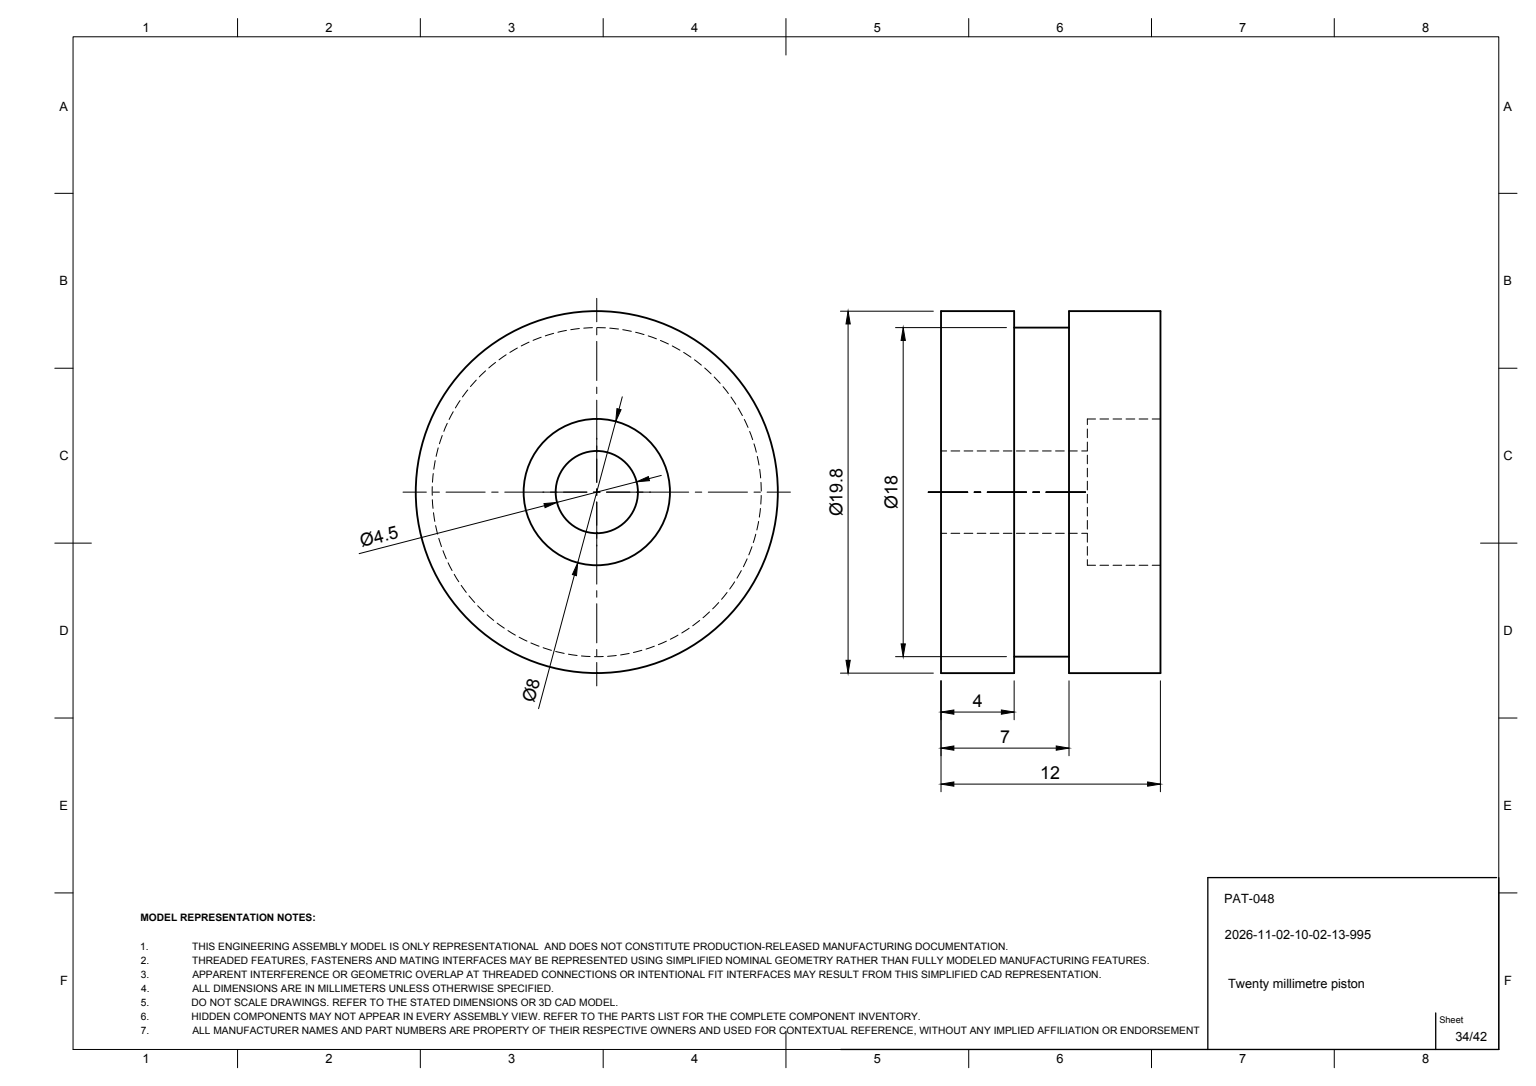
ISO-10303-21;
HEADER;
/* Generated by software containing ST-Developer
 * from STEP Tools, Inc. (www.steptools.com) 
 */

FILE_DESCRIPTION(
/* description */ ('Guided pneumatic stop gate'),
/* implementation_level */ '2;1');

FILE_NAME(
/* name */ 'Twenty millimetre piston.step',
/* time_stamp */ '2026-10-27T21:43:45-07:00',
/* author */ (''),
/* organization */ (''),
/* preprocessor_version */ 'ST-DEVELOPER v20.2',
/* originating_system */ 'Autodesk Translation Framework v15.17.0.0',
/* authorisation */ '');

FILE_SCHEMA (('AUTOMOTIVE_DESIGN { 1 0 10303 214 3 1 1 }'));
ENDSEC;

DATA;
#10=MECHANICAL_DESIGN_GEOMETRIC_PRESENTATION_REPRESENTATION('',(#563),#14392);
#479=SHAPE_REPRESENTATION_RELATIONSHIP('SRR','None',#14616,#521);
#521=ADVANCED_BREP_SHAPE_REPRESENTATION('',(#602),#14378);
#563=STYLED_ITEM('',(#14905),#602);
#602=MANIFOLD_SOLID_BREP('Body1',#7906);
#791=FACE_BOUND('',#2129,.T.);
#792=FACE_BOUND('',#2132,.T.);
#793=FACE_BOUND('',#2134,.T.);
#794=FACE_BOUND('',#2139,.T.);
#795=FACE_BOUND('',#2141,.T.);
#1043=PLANE('',#9159);
#1044=PLANE('',#9164);
#1045=PLANE('',#9166);
#1046=PLANE('',#9174);
#1047=PLANE('',#9175);
#1476=FACE_OUTER_BOUND('',#2127,.T.);
#1477=FACE_OUTER_BOUND('',#2128,.T.);
#1478=FACE_OUTER_BOUND('',#2130,.T.);
#1479=FACE_OUTER_BOUND('',#2131,.T.);
#1480=FACE_OUTER_BOUND('',#2133,.T.);
#1481=FACE_OUTER_BOUND('',#2135,.T.);
#1482=FACE_OUTER_BOUND('',#2136,.T.);
#1483=FACE_OUTER_BOUND('',#2137,.T.);
#1484=FACE_OUTER_BOUND('',#2138,.T.);
#1485=FACE_OUTER_BOUND('',#2140,.T.);
#2127=EDGE_LOOP('',(#6772,#6773,#6774,#6775));
#2128=EDGE_LOOP('',(#6776));
#2129=EDGE_LOOP('',(#6777));
#2130=EDGE_LOOP('',(#6778,#6779,#6780,#6781));
#2131=EDGE_LOOP('',(#6782));
#2132=EDGE_LOOP('',(#6783));
#2133=EDGE_LOOP('',(#6784));
#2134=EDGE_LOOP('',(#6785));
#2135=EDGE_LOOP('',(#6786,#6787,#6788,#6789));
#2136=EDGE_LOOP('',(#6790,#6791,#6792,#6793));
#2137=EDGE_LOOP('',(#6794,#6795,#6796,#6797));
#2138=EDGE_LOOP('',(#6798));
#2139=EDGE_LOOP('',(#6799));
#2140=EDGE_LOOP('',(#6800));
#2141=EDGE_LOOP('',(#6801));
#2686=LINE('',#13608,#3231);
#2687=LINE('',#13617,#3232);
#2688=LINE('',#13627,#3233);
#2689=LINE('',#13631,#3234);
#2690=LINE('',#13636,#3235);
#3231=VECTOR('',#11337,0.4);
#3232=VECTOR('',#11348,0.9);
#3233=VECTOR('',#11361,0.99);
#3234=VECTOR('',#11366,0.225);
#3235=VECTOR('',#11373,0.99);
#3662=CIRCLE('',#9157,0.4);
#3663=CIRCLE('',#9158,0.4);
#3664=CIRCLE('',#9160,0.225);
#3665=CIRCLE('',#9162,0.9);
#3666=CIRCLE('',#9163,0.9);
#3667=CIRCLE('',#9165,0.99);
#3668=CIRCLE('',#9167,0.99);
#3669=CIRCLE('',#9169,0.99);
#3670=CIRCLE('',#9171,0.225);
#3671=CIRCLE('',#9173,0.99);
#4205=VERTEX_POINT('',#13605);
#4206=VERTEX_POINT('',#13607);
#4207=VERTEX_POINT('',#13611);
#4208=VERTEX_POINT('',#13614);
#4209=VERTEX_POINT('',#13616);
#4210=VERTEX_POINT('',#13620);
#4211=VERTEX_POINT('',#13623);
#4212=VERTEX_POINT('',#13626);
#4213=VERTEX_POINT('',#13630);
#4214=VERTEX_POINT('',#13634);
#5084=EDGE_CURVE('',#4205,#4205,#3662,.T.);
#5085=EDGE_CURVE('',#4205,#4206,#2686,.T.);
#5086=EDGE_CURVE('',#4206,#4206,#3663,.T.);
#5087=EDGE_CURVE('',#4207,#4207,#3664,.T.);
#5088=EDGE_CURVE('',#4208,#4208,#3665,.T.);
#5089=EDGE_CURVE('',#4208,#4209,#2687,.T.);
#5090=EDGE_CURVE('',#4209,#4209,#3666,.T.);
#5091=EDGE_CURVE('',#4210,#4210,#3667,.T.);
#5092=EDGE_CURVE('',#4211,#4211,#3668,.T.);
#5093=EDGE_CURVE('',#4211,#4212,#2688,.T.);
#5094=EDGE_CURVE('',#4212,#4212,#3669,.T.);
#5095=EDGE_CURVE('',#4207,#4213,#2689,.T.);
#5096=EDGE_CURVE('',#4213,#4213,#3670,.T.);
#5097=EDGE_CURVE('',#4214,#4214,#3671,.T.);
#5098=EDGE_CURVE('',#4214,#4210,#2690,.T.);
#6772=ORIENTED_EDGE('',*,*,#5084,.F.);
#6773=ORIENTED_EDGE('',*,*,#5085,.T.);
#6774=ORIENTED_EDGE('',*,*,#5086,.F.);
#6775=ORIENTED_EDGE('',*,*,#5085,.F.);
#6776=ORIENTED_EDGE('',*,*,#5084,.T.);
#6777=ORIENTED_EDGE('',*,*,#5087,.F.);
#6778=ORIENTED_EDGE('',*,*,#5088,.F.);
#6779=ORIENTED_EDGE('',*,*,#5089,.T.);
#6780=ORIENTED_EDGE('',*,*,#5090,.T.);
#6781=ORIENTED_EDGE('',*,*,#5089,.F.);
#6782=ORIENTED_EDGE('',*,*,#5091,.F.);
#6783=ORIENTED_EDGE('',*,*,#5090,.F.);
#6784=ORIENTED_EDGE('',*,*,#5092,.F.);
#6785=ORIENTED_EDGE('',*,*,#5088,.T.);
#6786=ORIENTED_EDGE('',*,*,#5092,.T.);
#6787=ORIENTED_EDGE('',*,*,#5093,.T.);
#6788=ORIENTED_EDGE('',*,*,#5094,.T.);
#6789=ORIENTED_EDGE('',*,*,#5093,.F.);
#6790=ORIENTED_EDGE('',*,*,#5087,.T.);
#6791=ORIENTED_EDGE('',*,*,#5095,.T.);
#6792=ORIENTED_EDGE('',*,*,#5096,.T.);
#6793=ORIENTED_EDGE('',*,*,#5095,.F.);
#6794=ORIENTED_EDGE('',*,*,#5097,.F.);
#6795=ORIENTED_EDGE('',*,*,#5098,.T.);
#6796=ORIENTED_EDGE('',*,*,#5091,.T.);
#6797=ORIENTED_EDGE('',*,*,#5098,.F.);
#6798=ORIENTED_EDGE('',*,*,#5097,.T.);
#6799=ORIENTED_EDGE('',*,*,#5086,.T.);
#6800=ORIENTED_EDGE('',*,*,#5094,.F.);
#6801=ORIENTED_EDGE('',*,*,#5096,.F.);
#7370=CYLINDRICAL_SURFACE('',#9156,0.4);
#7371=CYLINDRICAL_SURFACE('',#9161,0.9);
#7372=CYLINDRICAL_SURFACE('',#9168,0.99);
#7373=CYLINDRICAL_SURFACE('',#9170,0.225);
#7374=CYLINDRICAL_SURFACE('',#9172,0.99);
#7758=ADVANCED_FACE('',(#1476),#7370,.F.);
#7759=ADVANCED_FACE('',(#1477,#791),#1043,.T.);
#7760=ADVANCED_FACE('',(#1478),#7371,.T.);
#7761=ADVANCED_FACE('',(#1479,#792),#1044,.F.);
#7762=ADVANCED_FACE('',(#1480,#793),#1045,.T.);
#7763=ADVANCED_FACE('',(#1481),#7372,.T.);
#7764=ADVANCED_FACE('',(#1482),#7373,.F.);
#7765=ADVANCED_FACE('',(#1483),#7374,.T.);
#7766=ADVANCED_FACE('',(#1484,#794),#1046,.T.);
#7767=ADVANCED_FACE('',(#1485,#795),#1047,.F.);
#7906=CLOSED_SHELL('',(#7758,#7759,#7760,#7761,#7762,#7763,#7764,#7765,
#7766,#7767));
#9155=AXIS2_PLACEMENT_3D('',#13603,#11331,#11332);
#9156=AXIS2_PLACEMENT_3D('',#13604,#11333,#11334);
#9157=AXIS2_PLACEMENT_3D('',#13606,#11335,#11336);
#9158=AXIS2_PLACEMENT_3D('',#13609,#11338,#11339);
#9159=AXIS2_PLACEMENT_3D('',#13610,#11340,#11341);
#9160=AXIS2_PLACEMENT_3D('',#13612,#11342,#11343);
#9161=AXIS2_PLACEMENT_3D('',#13613,#11344,#11345);
#9162=AXIS2_PLACEMENT_3D('',#13615,#11346,#11347);
#9163=AXIS2_PLACEMENT_3D('',#13618,#11349,#11350);
#9164=AXIS2_PLACEMENT_3D('',#13619,#11351,#11352);
#9165=AXIS2_PLACEMENT_3D('',#13621,#11353,#11354);
#9166=AXIS2_PLACEMENT_3D('',#13622,#11355,#11356);
#9167=AXIS2_PLACEMENT_3D('',#13624,#11357,#11358);
#9168=AXIS2_PLACEMENT_3D('',#13625,#11359,#11360);
#9169=AXIS2_PLACEMENT_3D('',#13628,#11362,#11363);
#9170=AXIS2_PLACEMENT_3D('',#13629,#11364,#11365);
#9171=AXIS2_PLACEMENT_3D('',#13632,#11367,#11368);
#9172=AXIS2_PLACEMENT_3D('',#13633,#11369,#11370);
#9173=AXIS2_PLACEMENT_3D('',#13635,#11371,#11372);
#9174=AXIS2_PLACEMENT_3D('',#13637,#11374,#11375);
#9175=AXIS2_PLACEMENT_3D('',#13638,#11376,#11377);
#11331=DIRECTION('axis',(0.,0.,1.));
#11332=DIRECTION('refdir',(1.,0.,0.));
#11333=DIRECTION('center_axis',(0.,1.,0.));
#11334=DIRECTION('ref_axis',(1.,0.,0.));
#11335=DIRECTION('center_axis',(0.,1.,0.));
#11336=DIRECTION('ref_axis',(1.,0.,0.));
#11337=DIRECTION('',(0.,1.,0.));
#11338=DIRECTION('center_axis',(0.,-1.,0.));
#11339=DIRECTION('ref_axis',(1.,0.,0.));
#11340=DIRECTION('center_axis',(0.,1.,0.));
#11341=DIRECTION('ref_axis',(1.,0.,0.));
#11342=DIRECTION('center_axis',(0.,1.,0.));
#11343=DIRECTION('ref_axis',(1.,0.,0.));
#11344=DIRECTION('center_axis',(0.,1.,0.));
#11345=DIRECTION('ref_axis',(1.,0.,0.));
#11346=DIRECTION('center_axis',(0.,-1.,0.));
#11347=DIRECTION('ref_axis',(1.,0.,0.));
#11348=DIRECTION('',(0.,1.,0.));
#11349=DIRECTION('center_axis',(0.,-1.,0.));
#11350=DIRECTION('ref_axis',(1.,0.,0.));
#11351=DIRECTION('center_axis',(0.,1.,0.));
#11352=DIRECTION('ref_axis',(1.,0.,0.));
#11353=DIRECTION('center_axis',(0.,1.,0.));
#11354=DIRECTION('ref_axis',(1.,0.,0.));
#11355=DIRECTION('center_axis',(0.,1.,0.));
#11356=DIRECTION('ref_axis',(1.,0.,0.));
#11357=DIRECTION('center_axis',(0.,-1.,0.));
#11358=DIRECTION('ref_axis',(1.,0.,0.));
#11359=DIRECTION('center_axis',(0.,1.,0.));
#11360=DIRECTION('ref_axis',(1.,0.,0.));
#11361=DIRECTION('',(0.,-1.,0.));
#11362=DIRECTION('center_axis',(0.,1.,0.));
#11363=DIRECTION('ref_axis',(1.,0.,0.));
#11364=DIRECTION('center_axis',(0.,1.,0.));
#11365=DIRECTION('ref_axis',(1.,0.,0.));
#11366=DIRECTION('',(0.,-1.,0.));
#11367=DIRECTION('center_axis',(0.,-1.,0.));
#11368=DIRECTION('ref_axis',(1.,0.,0.));
#11369=DIRECTION('center_axis',(0.,1.,0.));
#11370=DIRECTION('ref_axis',(1.,0.,0.));
#11371=DIRECTION('center_axis',(0.,1.,0.));
#11372=DIRECTION('ref_axis',(1.,0.,0.));
#11373=DIRECTION('',(0.,-1.,0.));
#11374=DIRECTION('center_axis',(0.,1.,0.));
#11375=DIRECTION('ref_axis',(1.,0.,0.));
#11376=DIRECTION('center_axis',(0.,1.,0.));
#11377=DIRECTION('ref_axis',(1.,0.,0.));
#13603=CARTESIAN_POINT('',(0.,0.,0.));
#13604=CARTESIAN_POINT('Origin',(0.,3.2,4.5));
#13605=CARTESIAN_POINT('',(-0.4,3.2,4.5));
#13606=CARTESIAN_POINT('Origin',(0.,3.2,4.5));
#13607=CARTESIAN_POINT('',(-0.4,3.6,4.5));
#13608=CARTESIAN_POINT('',(-0.4,3.2,4.5));
#13609=CARTESIAN_POINT('Origin',(0.,3.6,4.5));
#13610=CARTESIAN_POINT('Origin',(0.,3.2,4.5));
#13611=CARTESIAN_POINT('',(-0.225,3.2,4.5));
#13612=CARTESIAN_POINT('Origin',(0.,3.2,4.5));
#13613=CARTESIAN_POINT('Origin',(0.,2.8,4.5));
#13614=CARTESIAN_POINT('',(-0.9,2.8,4.5));
#13615=CARTESIAN_POINT('Origin',(0.,2.8,4.5));
#13616=CARTESIAN_POINT('',(-0.9,3.1,4.5));
#13617=CARTESIAN_POINT('',(-0.9,2.8,4.5));
#13618=CARTESIAN_POINT('Origin',(0.,3.1,4.5));
#13619=CARTESIAN_POINT('Origin',(0.,3.1,4.5));
#13620=CARTESIAN_POINT('',(-0.99,3.1,4.5));
#13621=CARTESIAN_POINT('Origin',(0.,3.1,4.5));
#13622=CARTESIAN_POINT('Origin',(0.,2.8,4.5));
#13623=CARTESIAN_POINT('',(-0.99,2.8,4.5));
#13624=CARTESIAN_POINT('Origin',(0.,2.8,4.5));
#13625=CARTESIAN_POINT('Origin',(0.,2.4,4.5));
#13626=CARTESIAN_POINT('',(-0.99,2.4,4.5));
#13627=CARTESIAN_POINT('',(-0.99,2.4,4.5));
#13628=CARTESIAN_POINT('Origin',(0.,2.4,4.5));
#13629=CARTESIAN_POINT('Origin',(0.,2.4,4.5));
#13630=CARTESIAN_POINT('',(-0.225,2.4,4.5));
#13631=CARTESIAN_POINT('',(-0.225,2.4,4.5));
#13632=CARTESIAN_POINT('Origin',(0.,2.4,4.5));
#13633=CARTESIAN_POINT('Origin',(0.,2.4,4.5));
#13634=CARTESIAN_POINT('',(-0.99,3.6,4.5));
#13635=CARTESIAN_POINT('Origin',(0.,3.6,4.5));
#13636=CARTESIAN_POINT('',(-0.99,2.4,4.5));
#13637=CARTESIAN_POINT('Origin',(0.,3.6,4.5));
#13638=CARTESIAN_POINT('Origin',(0.,2.4,4.5));
#14330=UNCERTAINTY_MEASURE_WITH_UNIT(LENGTH_MEASURE(0.001),#14393,
'DISTANCE_ACCURACY_VALUE',
'Maximum model space distance between geometric entities at asserted c
onnectivities');
#14344=UNCERTAINTY_MEASURE_WITH_UNIT(LENGTH_MEASURE(0.001),#14393,
'DISTANCE_ACCURACY_VALUE',
'Maximum model space distance between geometric entities at asserted c
onnectivities');
#14378=(
GEOMETRIC_REPRESENTATION_CONTEXT(3)
GLOBAL_UNCERTAINTY_ASSIGNED_CONTEXT((#14330))
GLOBAL_UNIT_ASSIGNED_CONTEXT((#14393,#14395,#14396))
REPRESENTATION_CONTEXT('','3D')
);
#14392=(
GEOMETRIC_REPRESENTATION_CONTEXT(3)
GLOBAL_UNCERTAINTY_ASSIGNED_CONTEXT((#14344))
GLOBAL_UNIT_ASSIGNED_CONTEXT((#14393,#14395,#14396))
REPRESENTATION_CONTEXT('','3D')
);
#14393=(
LENGTH_UNIT()
NAMED_UNIT(*)
SI_UNIT(.CENTI.,.METRE.)
);
#14395=(
NAMED_UNIT(*)
PLANE_ANGLE_UNIT()
SI_UNIT($,.RADIAN.)
);
#14396=(
NAMED_UNIT(*)
SI_UNIT($,.STERADIAN.)
SOLID_ANGLE_UNIT()
);
#14430=SHAPE_DEFINITION_REPRESENTATION(#14549,#14616);
#14549=PRODUCT_DEFINITION_SHAPE('',$,#14664);
#14616=SHAPE_REPRESENTATION('',(#9155),#14378);
#14630=PRODUCT_DEFINITION_CONTEXT('part definition',#14773,'design');
#14664=PRODUCT_DEFINITION('Twenty millimetre piston',
'Twenty millimetre piston',#14711,#14630);
#14711=PRODUCT_DEFINITION_FORMATION('',$,#14808);
#14773=APPLICATION_CONTEXT(
'Core Data for Automotive Mechanical Design Process');
#14774=PRODUCT_CONTEXT('part definition',#14773,'mechanical');
#14808=PRODUCT('Twenty millimetre piston','Twenty millimetre piston',
'Twenty millimetre piston',(#14774));
#14899=COLOUR_RGB('Off White',0.89,0.88,0.83);
#14900=FILL_AREA_STYLE_COLOUR('',#14899);
#14901=FILL_AREA_STYLE('',(#14900));
#14902=SURFACE_STYLE_FILL_AREA(#14901);
#14903=SURFACE_SIDE_STYLE('',(#14902));
#14904=SURFACE_STYLE_USAGE(.BOTH.,#14903);
#14905=PRESENTATION_STYLE_ASSIGNMENT((#14904));
ENDSEC;
END-ISO-10303-21;
